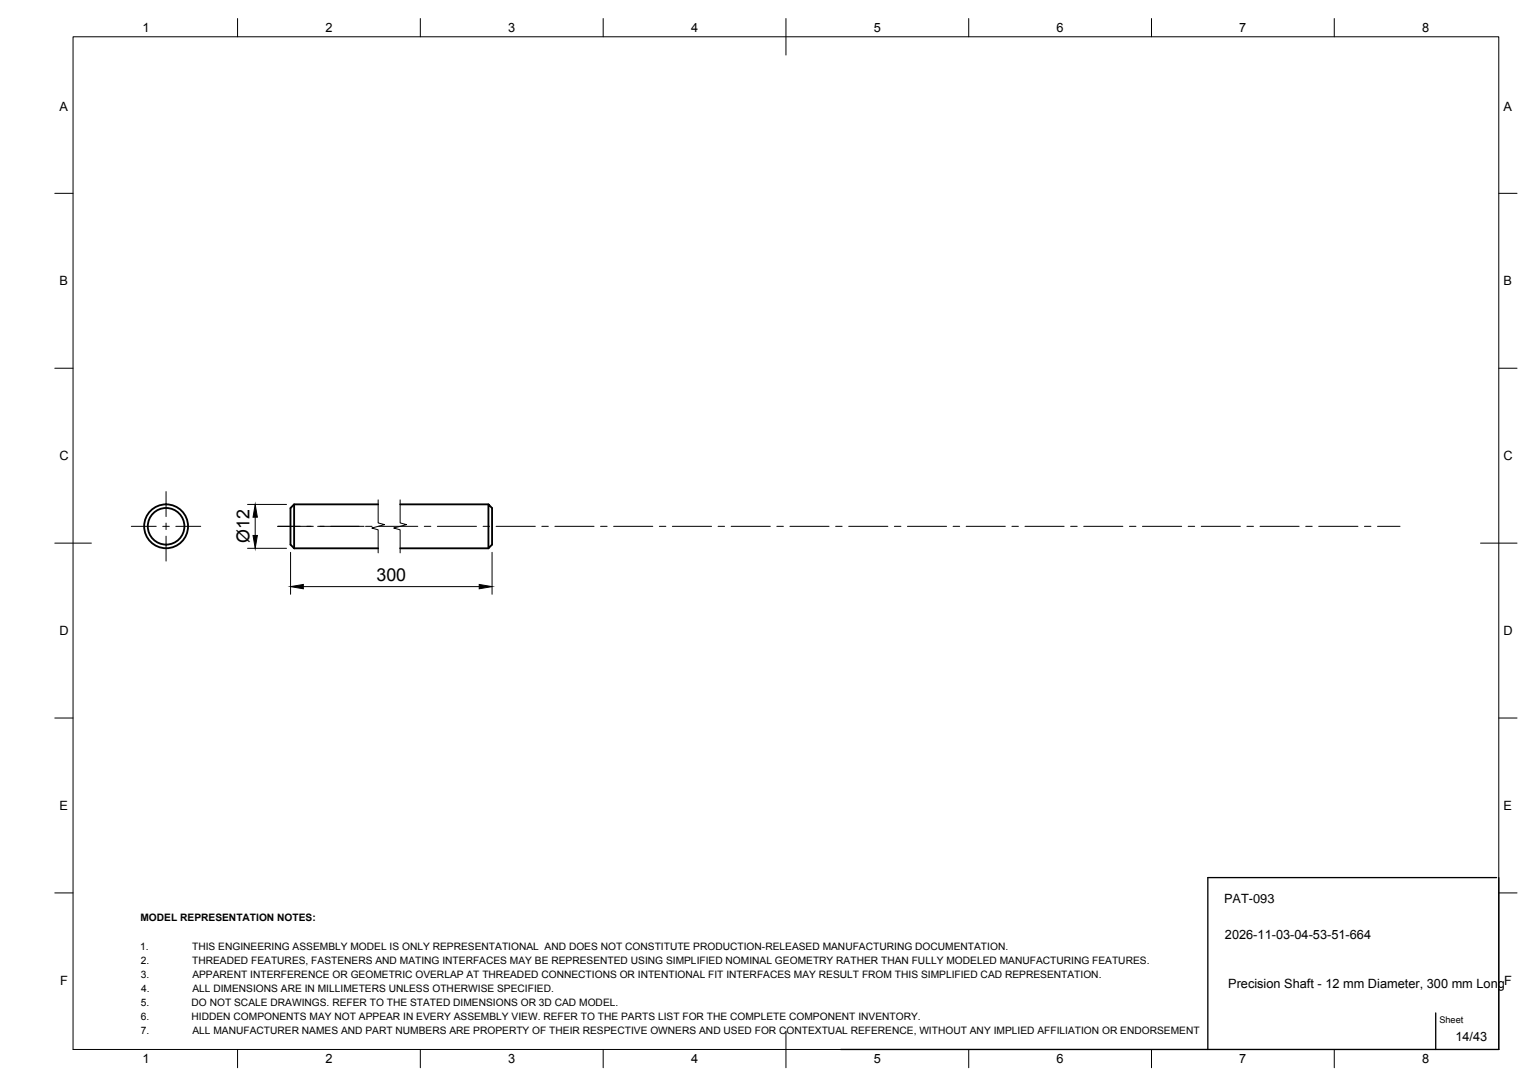
ISO-10303-21;
HEADER;
/* Generated by software containing ST-Developer
 * from STEP Tools, Inc. (www.steptools.com) 
 */

FILE_DESCRIPTION(
/* description */ ('Self-centering screw clamp'),
/* implementation_level */ '2;1');

FILE_NAME(
/* name */ 'Precision Shaft - 12 mm Diameter, 300 mm Long.step',
/* time_stamp */ '2026-10-28T03:25:31-07:00',
/* author */ (''),
/* organization */ (''),
/* preprocessor_version */ 'ST-DEVELOPER v20.2',
/* originating_system */ 'Autodesk Translation Framework v15.17.0.0',
/* authorisation */ '');

FILE_SCHEMA (('AUTOMOTIVE_DESIGN { 1 0 10303 214 3 1 1 }'));
ENDSEC;

DATA;
#10=MECHANICAL_DESIGN_GEOMETRIC_PRESENTATION_REPRESENTATION('',(#637),#16799);
#483=CONICAL_SURFACE('',#9945,0.55,0.785398163397448);
#484=CONICAL_SURFACE('',#9951,0.55,0.785398163397441);
#555=SHAPE_REPRESENTATION_RELATIONSHIP('SRR','None',#17028,#596);
#596=ADVANCED_BREP_SHAPE_REPRESENTATION('',(#685),#16766);
#637=STYLED_ITEM('',(#17326),#685);
#685=MANIFOLD_SOLID_BREP('Body1',#9088);
#1104=PLANE('',#9950);
#1105=PLANE('',#9953);
#1449=FACE_OUTER_BOUND('',#2077,.T.);
#1450=FACE_OUTER_BOUND('',#2078,.T.);
#1451=FACE_OUTER_BOUND('',#2079,.T.);
#1452=FACE_OUTER_BOUND('',#2080,.T.);
#1453=FACE_OUTER_BOUND('',#2081,.T.);
#2077=EDGE_LOOP('',(#6979,#6980,#6981,#6982));
#2078=EDGE_LOOP('',(#6983,#6984,#6985,#6986));
#2079=EDGE_LOOP('',(#6987));
#2080=EDGE_LOOP('',(#6988,#6989,#6990,#6991));
#2081=EDGE_LOOP('',(#6992));
#2823=LINE('',#14669,#3396);
#2824=LINE('',#14674,#3397);
#2825=LINE('',#14679,#3398);
#3396=VECTOR('',#11738,0.55);
#3397=VECTOR('',#11745,0.6);
#3398=VECTOR('',#11752,0.55);
#3899=CIRCLE('',#9946,0.6);
#3900=CIRCLE('',#9947,0.5);
#3901=CIRCLE('',#9949,0.6);
#3902=CIRCLE('',#9952,0.5);
#4513=VERTEX_POINT('',#14666);
#4514=VERTEX_POINT('',#14668);
#4515=VERTEX_POINT('',#14672);
#4516=VERTEX_POINT('',#14677);
#5414=EDGE_CURVE('',#4513,#4513,#3899,.T.);
#5415=EDGE_CURVE('',#4513,#4514,#2823,.T.);
#5416=EDGE_CURVE('',#4514,#4514,#3900,.T.);
#5417=EDGE_CURVE('',#4515,#4515,#3901,.T.);
#5418=EDGE_CURVE('',#4515,#4513,#2824,.T.);
#5419=EDGE_CURVE('',#4516,#4516,#3902,.T.);
#5420=EDGE_CURVE('',#4516,#4515,#2825,.T.);
#6979=ORIENTED_EDGE('',*,*,#5414,.T.);
#6980=ORIENTED_EDGE('',*,*,#5415,.T.);
#6981=ORIENTED_EDGE('',*,*,#5416,.T.);
#6982=ORIENTED_EDGE('',*,*,#5415,.F.);
#6983=ORIENTED_EDGE('',*,*,#5417,.F.);
#6984=ORIENTED_EDGE('',*,*,#5418,.T.);
#6985=ORIENTED_EDGE('',*,*,#5414,.F.);
#6986=ORIENTED_EDGE('',*,*,#5418,.F.);
#6987=ORIENTED_EDGE('',*,*,#5416,.F.);
#6988=ORIENTED_EDGE('',*,*,#5419,.T.);
#6989=ORIENTED_EDGE('',*,*,#5420,.T.);
#6990=ORIENTED_EDGE('',*,*,#5417,.T.);
#6991=ORIENTED_EDGE('',*,*,#5420,.F.);
#6992=ORIENTED_EDGE('',*,*,#5419,.F.);
#8443=CYLINDRICAL_SURFACE('',#9948,0.6);
#8747=ADVANCED_FACE('',(#1449),#483,.T.);
#8748=ADVANCED_FACE('',(#1450),#8443,.T.);
#8749=ADVANCED_FACE('',(#1451),#1104,.F.);
#8750=ADVANCED_FACE('',(#1452),#484,.T.);
#8751=ADVANCED_FACE('',(#1453),#1105,.T.);
#9088=CLOSED_SHELL('',(#8747,#8748,#8749,#8750,#8751));
#9944=AXIS2_PLACEMENT_3D('',#14664,#11732,#11733);
#9945=AXIS2_PLACEMENT_3D('',#14665,#11734,#11735);
#9946=AXIS2_PLACEMENT_3D('',#14667,#11736,#11737);
#9947=AXIS2_PLACEMENT_3D('',#14670,#11739,#11740);
#9948=AXIS2_PLACEMENT_3D('',#14671,#11741,#11742);
#9949=AXIS2_PLACEMENT_3D('',#14673,#11743,#11744);
#9950=AXIS2_PLACEMENT_3D('',#14675,#11746,#11747);
#9951=AXIS2_PLACEMENT_3D('',#14676,#11748,#11749);
#9952=AXIS2_PLACEMENT_3D('',#14678,#11750,#11751);
#9953=AXIS2_PLACEMENT_3D('',#14680,#11753,#11754);
#11732=DIRECTION('axis',(0.,0.,1.));
#11733=DIRECTION('refdir',(1.,0.,0.));
#11734=DIRECTION('center_axis',(1.,0.,0.));
#11735=DIRECTION('ref_axis',(0.,0.,-1.));
#11736=DIRECTION('center_axis',(-1.,0.,0.));
#11737=DIRECTION('ref_axis',(0.,0.,-1.));
#11738=DIRECTION('',(-0.707106781186548,8.65956056235493E-17,-0.707106781186547));
#11739=DIRECTION('center_axis',(1.,0.,0.));
#11740=DIRECTION('ref_axis',(0.,0.,-1.));
#11741=DIRECTION('center_axis',(1.,0.,0.));
#11742=DIRECTION('ref_axis',(0.,0.,-1.));
#11743=DIRECTION('center_axis',(1.,0.,0.));
#11744=DIRECTION('ref_axis',(0.,0.,-1.));
#11745=DIRECTION('',(-1.,0.,0.));
#11746=DIRECTION('center_axis',(1.,0.,0.));
#11747=DIRECTION('ref_axis',(0.,0.,-1.));
#11748=DIRECTION('center_axis',(-1.,0.,0.));
#11749=DIRECTION('ref_axis',(0.,0.,-1.));
#11750=DIRECTION('center_axis',(-1.,0.,0.));
#11751=DIRECTION('ref_axis',(0.,0.,-1.));
#11752=DIRECTION('',(-0.707106781186553,-8.65956056235487E-17,0.707106781186542));
#11753=DIRECTION('center_axis',(1.,0.,0.));
#11754=DIRECTION('ref_axis',(0.,0.,-1.));
#14664=CARTESIAN_POINT('',(0.,0.,0.));
#14665=CARTESIAN_POINT('Origin',(0.05,0.,0.));
#14666=CARTESIAN_POINT('',(0.1,7.34788079488412E-17,0.6));
#14667=CARTESIAN_POINT('Origin',(0.1,0.,0.));
#14668=CARTESIAN_POINT('',(0.,-6.12323399573677E-17,0.5));
#14669=CARTESIAN_POINT('',(0.05,-6.73555739531044E-17,0.55));
#14670=CARTESIAN_POINT('Origin',(0.,0.,0.));
#14671=CARTESIAN_POINT('Origin',(0.,0.,0.));
#14672=CARTESIAN_POINT('',(29.9,-7.34788079488412E-17,0.6));
#14673=CARTESIAN_POINT('Origin',(29.9,0.,0.));
#14674=CARTESIAN_POINT('',(0.,-7.34788079488412E-17,0.6));
#14675=CARTESIAN_POINT('Origin',(0.,0.,0.));
#14676=CARTESIAN_POINT('Origin',(29.95,0.,0.));
#14677=CARTESIAN_POINT('',(30.,6.12323399573677E-17,0.5));
#14678=CARTESIAN_POINT('Origin',(30.,0.,0.));
#14679=CARTESIAN_POINT('',(29.95,-6.73555739531044E-17,0.55));
#14680=CARTESIAN_POINT('Origin',(30.,0.,0.));
#16717=UNCERTAINTY_MEASURE_WITH_UNIT(LENGTH_MEASURE(0.001),#16800,
'DISTANCE_ACCURACY_VALUE',
'Maximum model space distance between geometric entities at asserted c
onnectivities');
#16750=UNCERTAINTY_MEASURE_WITH_UNIT(LENGTH_MEASURE(0.001),#16800,
'DISTANCE_ACCURACY_VALUE',
'Maximum model space distance between geometric entities at asserted c
onnectivities');
#16766=(
GEOMETRIC_REPRESENTATION_CONTEXT(3)
GLOBAL_UNCERTAINTY_ASSIGNED_CONTEXT((#16717))
GLOBAL_UNIT_ASSIGNED_CONTEXT((#16800,#16802,#16803))
REPRESENTATION_CONTEXT('','3D')
);
#16799=(
GEOMETRIC_REPRESENTATION_CONTEXT(3)
GLOBAL_UNCERTAINTY_ASSIGNED_CONTEXT((#16750))
GLOBAL_UNIT_ASSIGNED_CONTEXT((#16800,#16802,#16803))
REPRESENTATION_CONTEXT('','3D')
);
#16800=(
LENGTH_UNIT()
NAMED_UNIT(*)
SI_UNIT(.CENTI.,.METRE.)
);
#16802=(
NAMED_UNIT(*)
PLANE_ANGLE_UNIT()
SI_UNIT($,.RADIAN.)
);
#16803=(
NAMED_UNIT(*)
SI_UNIT($,.STERADIAN.)
SOLID_ANGLE_UNIT()
);
#16819=SHAPE_DEFINITION_REPRESENTATION(#16867,#17028);
#16867=PRODUCT_DEFINITION_SHAPE('',$,#17077);
#17028=SHAPE_REPRESENTATION('',(#9944),#16766);
#17061=PRODUCT_DEFINITION_CONTEXT('part definition',#17207,'design');
#17077=PRODUCT_DEFINITION(
'Precision Shaft - 12 mm Diameter, 300 mm Long',
'Precision Shaft - 12 mm Diameter, 300 mm Long',#17125,#17061);
#17125=PRODUCT_DEFINITION_FORMATION('',$,#17224);
#17207=APPLICATION_CONTEXT(
'Core Data for Automotive Mechanical Design Process');
#17208=PRODUCT_CONTEXT('part definition',#17207,'mechanical');
#17224=PRODUCT('Precision Shaft - 12 mm Diameter, 300 mm Long',
'Precision Shaft - 12 mm Diameter, 300 mm Long',
'Precision Shaft - 12 mm Diameter, 300 mm Long',(#17208));
#17320=COLOUR_RGB('Grey',0.48,0.52,0.57);
#17321=FILL_AREA_STYLE_COLOUR('',#17320);
#17322=FILL_AREA_STYLE('',(#17321));
#17323=SURFACE_STYLE_FILL_AREA(#17322);
#17324=SURFACE_SIDE_STYLE('',(#17323));
#17325=SURFACE_STYLE_USAGE(.BOTH.,#17324);
#17326=PRESENTATION_STYLE_ASSIGNMENT((#17325));
ENDSEC;
END-ISO-10303-21;
